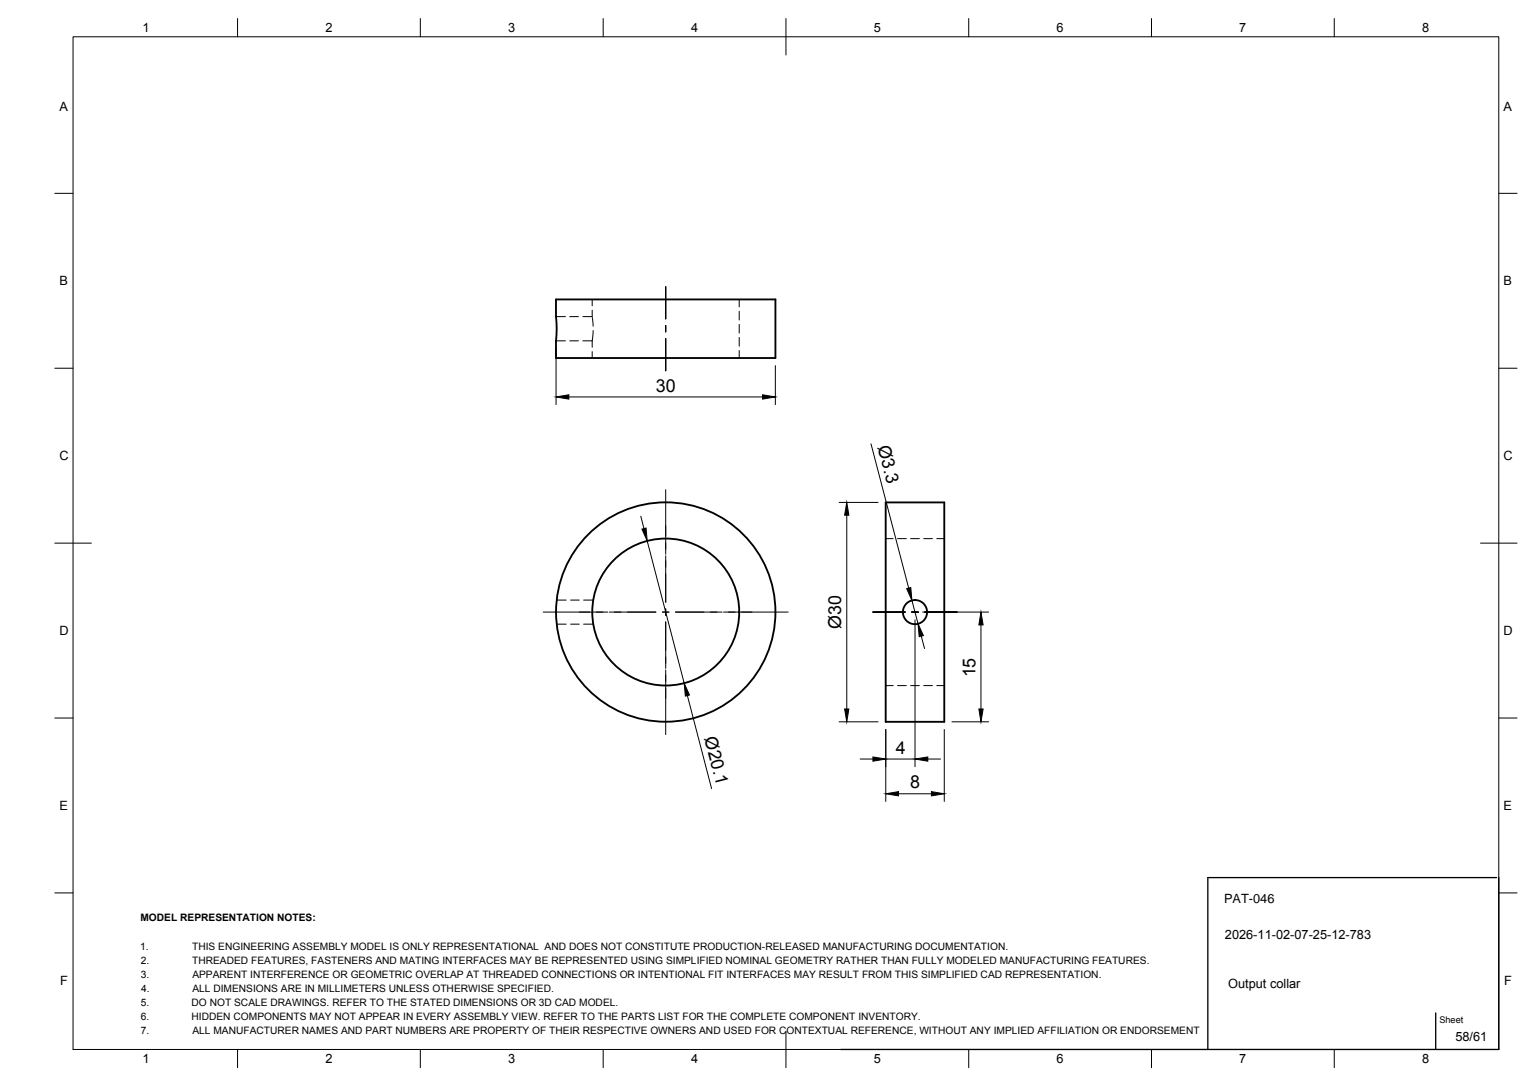
ISO-10303-21;
HEADER;
/* Generated by software containing ST-Developer
 * from STEP Tools, Inc. (www.steptools.com) 
 */

FILE_DESCRIPTION(
/* description */ ('Gear mesh backlash fixture'),
/* implementation_level */ '2;1');

FILE_NAME(
/* name */ 'Output collar.step',
/* time_stamp */ '2026-10-28T03:26:00-07:00',
/* author */ (''),
/* organization */ (''),
/* preprocessor_version */ 'ST-DEVELOPER v20.2',
/* originating_system */ 'Autodesk Translation Framework v15.17.0.0',
/* authorisation */ '');

FILE_SCHEMA (('AUTOMOTIVE_DESIGN { 1 0 10303 214 3 1 1 }'));
ENDSEC;

DATA;
#10=MECHANICAL_DESIGN_GEOMETRIC_PRESENTATION_REPRESENTATION('',(#1075),#57900);
#832=B_SPLINE_CURVE_WITH_KNOTS('',3,(#33907,#33908,#33909,#33910,#33911,
#33912,#33913,#33914,#33915,#33916),.UNSPECIFIED.,.F.,.F.,(4,2,2,2,4),(0.,
0.0622753849594661,0.124550769918932,0.186824589898798,0.249098409878664),
 .UNSPECIFIED.);
#833=B_SPLINE_CURVE_WITH_KNOTS('',3,(#33917,#33918,#33919,#33920,#33921,
#33922,#33923,#33924,#33925,#33926,#33927,#33928,#33929,#33930,#33931,#33932,
#33933,#33934,#33935,#33936,#33937,#33938,#33939,#33940,#33941,#33942),
 .UNSPECIFIED.,.F.,.F.,(4,2,2,2,2,2,2,2,2,2,2,2,4),(0.249098409878664,0.31137222985853,
0.373646049838396,0.435921434797862,0.498196819757329,0.560472204716795,
0.622747589676261,0.685021409656127,0.747295229635993,0.809569049615859,
0.871842869595725,0.934118254555191,0.996393639514657),.UNSPECIFIED.);
#834=B_SPLINE_CURVE_WITH_KNOTS('',3,(#33946,#33947,#33948,#33949,#33950,
#33951,#33952,#33953,#33954,#33955,#33956,#33957,#33958,#33959,#33960,#33961,
#33962,#33963,#33964,#33965,#33966,#33967,#33968,#33969,#33970,#33971),
 .UNSPECIFIED.,.F.,.F.,(4,2,2,2,2,2,2,2,2,2,2,2,4),(0.,0.0622075173149515,
0.124415034629903,0.186622241324509,0.248829448019115,0.311036654713721,
0.373243861408327,0.435451378723279,0.49765889603823,0.559866413353181,
0.622073930668133,0.684281137362739,0.746488344057345),.UNSPECIFIED.);
#835=B_SPLINE_CURVE_WITH_KNOTS('',3,(#33972,#33973,#33974,#33975,#33976,
#33977,#33978,#33979,#33980,#33981),.UNSPECIFIED.,.F.,.F.,(4,2,2,2,4),(0.746488344057345,
0.808695550751951,0.870902757446557,0.933110274761508,0.99531779207646),
 .UNSPECIFIED.);
#960=SHAPE_REPRESENTATION_RELATIONSHIP('SRR','None',#58161,#1010);
#1010=ADVANCED_BREP_SHAPE_REPRESENTATION('',(#1138),#57894);
#1075=STYLED_ITEM('',(#58479),#1138);
#1138=MANIFOLD_SOLID_BREP('Body1',#13637);
#1319=FACE_BOUND('',#3192,.T.);
#1320=FACE_BOUND('',#3194,.T.);
#1321=FACE_BOUND('',#3196,.T.);
#1322=FACE_BOUND('',#3198,.T.);
#1618=PLANE('',#15273);
#1619=PLANE('',#15274);
#2249=FACE_OUTER_BOUND('',#3190,.T.);
#2250=FACE_OUTER_BOUND('',#3191,.T.);
#2251=FACE_OUTER_BOUND('',#3193,.T.);
#2252=FACE_OUTER_BOUND('',#3195,.T.);
#2253=FACE_OUTER_BOUND('',#3197,.T.);
#3190=EDGE_LOOP('',(#11431,#11432,#11433,#11434,#11435,#11436));
#3191=EDGE_LOOP('',(#11437,#11438,#11439,#11440));
#3192=EDGE_LOOP('',(#11441,#11442));
#3193=EDGE_LOOP('',(#11443,#11444,#11445,#11446));
#3194=EDGE_LOOP('',(#11447,#11448));
#3195=EDGE_LOOP('',(#11449));
#3196=EDGE_LOOP('',(#11450));
#3197=EDGE_LOOP('',(#11451));
#3198=EDGE_LOOP('',(#11452));
#4069=LINE('',#33944,#4958);
#4070=LINE('',#33986,#4959);
#4071=LINE('',#33992,#4960);
#4958=VECTOR('',#18380,0.165);
#4959=VECTOR('',#18385,1.005);
#4960=VECTOR('',#18392,1.5);
#5679=CIRCLE('',#15268,1.005);
#5680=CIRCLE('',#15269,1.005);
#5681=CIRCLE('',#15271,1.5);
#5682=CIRCLE('',#15272,1.5);
#6642=VERTEX_POINT('',#33905);
#6643=VERTEX_POINT('',#33906);
#6644=VERTEX_POINT('',#33943);
#6645=VERTEX_POINT('',#33945);
#6646=VERTEX_POINT('',#33983);
#6647=VERTEX_POINT('',#33985);
#6648=VERTEX_POINT('',#33989);
#6649=VERTEX_POINT('',#33991);
#8302=EDGE_CURVE('',#6642,#6643,#832,.T.);
#8303=EDGE_CURVE('',#6643,#6642,#833,.T.);
#8304=EDGE_CURVE('',#6643,#6644,#4069,.T.);
#8305=EDGE_CURVE('',#6645,#6644,#834,.T.);
#8306=EDGE_CURVE('',#6644,#6645,#835,.T.);
#8307=EDGE_CURVE('',#6646,#6646,#5679,.T.);
#8308=EDGE_CURVE('',#6646,#6647,#4070,.T.);
#8309=EDGE_CURVE('',#6647,#6647,#5680,.T.);
#8310=EDGE_CURVE('',#6648,#6648,#5681,.T.);
#8311=EDGE_CURVE('',#6648,#6649,#4071,.T.);
#8312=EDGE_CURVE('',#6649,#6649,#5682,.T.);
#11431=ORIENTED_EDGE('',*,*,#8302,.F.);
#11432=ORIENTED_EDGE('',*,*,#8303,.F.);
#11433=ORIENTED_EDGE('',*,*,#8304,.T.);
#11434=ORIENTED_EDGE('',*,*,#8305,.F.);
#11435=ORIENTED_EDGE('',*,*,#8306,.F.);
#11436=ORIENTED_EDGE('',*,*,#8304,.F.);
#11437=ORIENTED_EDGE('',*,*,#8307,.F.);
#11438=ORIENTED_EDGE('',*,*,#8308,.T.);
#11439=ORIENTED_EDGE('',*,*,#8309,.T.);
#11440=ORIENTED_EDGE('',*,*,#8308,.F.);
#11441=ORIENTED_EDGE('',*,*,#8302,.T.);
#11442=ORIENTED_EDGE('',*,*,#8303,.T.);
#11443=ORIENTED_EDGE('',*,*,#8310,.F.);
#11444=ORIENTED_EDGE('',*,*,#8311,.T.);
#11445=ORIENTED_EDGE('',*,*,#8312,.T.);
#11446=ORIENTED_EDGE('',*,*,#8311,.F.);
#11447=ORIENTED_EDGE('',*,*,#8305,.T.);
#11448=ORIENTED_EDGE('',*,*,#8306,.T.);
#11449=ORIENTED_EDGE('',*,*,#8310,.T.);
#11450=ORIENTED_EDGE('',*,*,#8307,.T.);
#11451=ORIENTED_EDGE('',*,*,#8312,.F.);
#11452=ORIENTED_EDGE('',*,*,#8309,.F.);
#12761=CYLINDRICAL_SURFACE('',#15266,0.165);
#12762=CYLINDRICAL_SURFACE('',#15267,1.005);
#12763=CYLINDRICAL_SURFACE('',#15270,1.5);
#13366=ADVANCED_FACE('',(#2249),#12761,.F.);
#13367=ADVANCED_FACE('',(#2250,#1319),#12762,.F.);
#13368=ADVANCED_FACE('',(#2251,#1320),#12763,.T.);
#13369=ADVANCED_FACE('',(#2252,#1321),#1618,.T.);
#13370=ADVANCED_FACE('',(#2253,#1322),#1619,.F.);
#13637=CLOSED_SHELL('',(#13366,#13367,#13368,#13369,#13370));
#15265=AXIS2_PLACEMENT_3D('',#33903,#18376,#18377);
#15266=AXIS2_PLACEMENT_3D('',#33904,#18378,#18379);
#15267=AXIS2_PLACEMENT_3D('',#33982,#18381,#18382);
#15268=AXIS2_PLACEMENT_3D('',#33984,#18383,#18384);
#15269=AXIS2_PLACEMENT_3D('',#33987,#18386,#18387);
#15270=AXIS2_PLACEMENT_3D('',#33988,#18388,#18389);
#15271=AXIS2_PLACEMENT_3D('',#33990,#18390,#18391);
#15272=AXIS2_PLACEMENT_3D('',#33993,#18393,#18394);
#15273=AXIS2_PLACEMENT_3D('',#33994,#18395,#18396);
#15274=AXIS2_PLACEMENT_3D('',#33995,#18397,#18398);
#18376=DIRECTION('axis',(0.,0.,1.));
#18377=DIRECTION('refdir',(1.,0.,0.));
#18378=DIRECTION('center_axis',(1.,0.,0.));
#18379=DIRECTION('ref_axis',(0.,0.,-1.));
#18380=DIRECTION('',(1.,0.,0.));
#18381=DIRECTION('center_axis',(0.,0.,1.));
#18382=DIRECTION('ref_axis',(1.,0.,0.));
#18383=DIRECTION('center_axis',(0.,0.,-1.));
#18384=DIRECTION('ref_axis',(1.,0.,0.));
#18385=DIRECTION('',(0.,0.,-1.));
#18386=DIRECTION('center_axis',(0.,0.,-1.));
#18387=DIRECTION('ref_axis',(1.,0.,0.));
#18388=DIRECTION('center_axis',(0.,0.,1.));
#18389=DIRECTION('ref_axis',(1.,0.,0.));
#18390=DIRECTION('center_axis',(0.,0.,1.));
#18391=DIRECTION('ref_axis',(1.,0.,0.));
#18392=DIRECTION('',(0.,0.,-1.));
#18393=DIRECTION('center_axis',(0.,0.,1.));
#18394=DIRECTION('ref_axis',(1.,0.,0.));
#18395=DIRECTION('center_axis',(0.,0.,1.));
#18396=DIRECTION('ref_axis',(1.,0.,0.));
#18397=DIRECTION('center_axis',(0.,0.,1.));
#18398=DIRECTION('ref_axis',(1.,0.,0.));
#33903=CARTESIAN_POINT('',(0.,0.,0.));
#33904=CARTESIAN_POINT('Origin',(6.99,0.,5.4));
#33905=CARTESIAN_POINT('',(6.9913626985115,0.165,5.4));
#33906=CARTESIAN_POINT('',(7.005,-1.18380595689425E-17,5.565));
#33907=CARTESIAN_POINT('Ctrl Pts',(6.9913626985115,0.165,5.4));
#33908=CARTESIAN_POINT('Ctrl Pts',(6.9913626985115,0.165,5.42075846165316));
#33909=CARTESIAN_POINT('Ctrl Pts',(6.99208213234536,0.160843707720237,5.44287436269219));
#33910=CARTESIAN_POINT('Ctrl Pts',(6.99466757507705,0.143993298000807,5.48351551009448));
#33911=CARTESIAN_POINT('Ctrl Pts',(6.9964948147884,0.131301190829395,5.50204404696217));
#33912=CARTESIAN_POINT('Ctrl Pts',(6.99991441892026,0.102044414577984,5.53130082321358));
#33913=CARTESIAN_POINT('Ctrl Pts',(7.00173085232892,0.083515719765581,5.54399321874371));
#33914=CARTESIAN_POINT('Ctrl Pts',(7.00429148829838,0.0428740302308134,
5.56084383788794));
#33915=CARTESIAN_POINT('Ctrl Pts',(7.005,0.0207579399932887,5.565));
#33916=CARTESIAN_POINT('Ctrl Pts',(7.005,2.60208521396521E-17,5.565));
#33917=CARTESIAN_POINT('Ctrl Pts',(7.005,-2.08166817117217E-17,5.565));
#33918=CARTESIAN_POINT('Ctrl Pts',(7.005,-0.0207579399932887,5.565));
#33919=CARTESIAN_POINT('Ctrl Pts',(7.00429148829838,-0.0428740302308134,
5.56084383788794));
#33920=CARTESIAN_POINT('Ctrl Pts',(7.00173085232892,-0.083515719765581,
5.54399321874371));
#33921=CARTESIAN_POINT('Ctrl Pts',(6.99991441892026,-0.102044414577984,
5.53130082321358));
#33922=CARTESIAN_POINT('Ctrl Pts',(6.9964948147884,-0.131301190829395,5.50204404696217));
#33923=CARTESIAN_POINT('Ctrl Pts',(6.99466757507705,-0.143993298000807,
5.48351551009448));
#33924=CARTESIAN_POINT('Ctrl Pts',(6.99208213234536,-0.160843707720237,
5.44287436269219));
#33925=CARTESIAN_POINT('Ctrl Pts',(6.9913626985115,-0.165,5.42075846165316));
#33926=CARTESIAN_POINT('Ctrl Pts',(6.9913626985115,-0.165,5.37924153834684));
#33927=CARTESIAN_POINT('Ctrl Pts',(6.99208213234536,-0.160843707720237,
5.35712563730781));
#33928=CARTESIAN_POINT('Ctrl Pts',(6.99466757507705,-0.143993298000807,
5.31648448990552));
#33929=CARTESIAN_POINT('Ctrl Pts',(6.9964948147884,-0.131301190829395,5.29795595303784));
#33930=CARTESIAN_POINT('Ctrl Pts',(6.99991441892026,-0.102044414577984,
5.26869917678642));
#33931=CARTESIAN_POINT('Ctrl Pts',(7.00173085232892,-0.083515719765581,
5.25600678125629));
#33932=CARTESIAN_POINT('Ctrl Pts',(7.00429148829838,-0.0428740302308134,
5.23915616211206));
#33933=CARTESIAN_POINT('Ctrl Pts',(7.005,-0.0207579399932887,5.235));
#33934=CARTESIAN_POINT('Ctrl Pts',(7.005,0.0207579399932886,5.235));
#33935=CARTESIAN_POINT('Ctrl Pts',(7.00429148829838,0.0428740302308133,
5.23915616211206));
#33936=CARTESIAN_POINT('Ctrl Pts',(7.00173085232892,0.0835157197655809,
5.25600678125629));
#33937=CARTESIAN_POINT('Ctrl Pts',(6.99991441892026,0.102044414577984,5.26869917678642));
#33938=CARTESIAN_POINT('Ctrl Pts',(6.9964948147884,0.131301190829395,5.29795595303784));
#33939=CARTESIAN_POINT('Ctrl Pts',(6.99466757507705,0.143993298000807,5.31648448990552));
#33940=CARTESIAN_POINT('Ctrl Pts',(6.99208213234536,0.160843707720237,5.35712563730781));
#33941=CARTESIAN_POINT('Ctrl Pts',(6.9913626985115,0.165,5.37924153834685));
#33942=CARTESIAN_POINT('Ctrl Pts',(6.9913626985115,0.165,5.4));
#33943=CARTESIAN_POINT('',(7.5,-2.02066721859313E-17,5.565));
#33944=CARTESIAN_POINT('',(6.99,-2.02066721859313E-17,5.565));
#33945=CARTESIAN_POINT('',(7.49089738077441,0.165,5.4));
#33946=CARTESIAN_POINT('Ctrl Pts',(7.49089738077441,0.165,5.4));
#33947=CARTESIAN_POINT('Ctrl Pts',(7.49089738077441,0.165,5.37926416089502));
#33948=CARTESIAN_POINT('Ctrl Pts',(7.49137458218466,0.160852499025072,5.35715772909914));
#33949=CARTESIAN_POINT('Ctrl Pts',(7.49309518705251,0.144008447160945,5.31651015506895));
#33950=CARTESIAN_POINT('Ctrl Pts',(7.49431341615514,0.131312810193433,5.29796757240187));
#33951=CARTESIAN_POINT('Ctrl Pts',(7.49659781052538,0.102032500700889,5.26868726290933));
#33952=CARTESIAN_POINT('Ctrl Pts',(7.49781281581157,0.0834898860986566,
5.25599156878035));
#33953=CARTESIAN_POINT('Ctrl Pts',(7.49952603771524,0.042842204593242,5.2391474746158));
#33954=CARTESIAN_POINT('Ctrl Pts',(7.5,0.0207357355648687,5.235));
#33955=CARTESIAN_POINT('Ctrl Pts',(7.5,-0.0207357355648687,5.235));
#33956=CARTESIAN_POINT('Ctrl Pts',(7.49952603771524,-0.042842204593242,
5.2391474746158));
#33957=CARTESIAN_POINT('Ctrl Pts',(7.49781281581157,-0.0834898860986566,
5.25599156878035));
#33958=CARTESIAN_POINT('Ctrl Pts',(7.49659781052538,-0.102032500700889,
5.26868726290933));
#33959=CARTESIAN_POINT('Ctrl Pts',(7.49431341615514,-0.131312810193433,
5.29796757240187));
#33960=CARTESIAN_POINT('Ctrl Pts',(7.49309518705251,-0.144008447160945,
5.31651015506895));
#33961=CARTESIAN_POINT('Ctrl Pts',(7.49137458218466,-0.160852499025072,
5.35715772909914));
#33962=CARTESIAN_POINT('Ctrl Pts',(7.49089738077441,-0.165,5.37926416089502));
#33963=CARTESIAN_POINT('Ctrl Pts',(7.49089738077441,-0.165,5.42073583910498));
#33964=CARTESIAN_POINT('Ctrl Pts',(7.49137458218466,-0.160852499025072,
5.44284227090086));
#33965=CARTESIAN_POINT('Ctrl Pts',(7.49309518705251,-0.144008447160945,
5.48348984493105));
#33966=CARTESIAN_POINT('Ctrl Pts',(7.49431341615514,-0.131312810193433,
5.50203242759813));
#33967=CARTESIAN_POINT('Ctrl Pts',(7.49659781052538,-0.102032500700889,
5.53131273709067));
#33968=CARTESIAN_POINT('Ctrl Pts',(7.49781281581157,-0.0834898860986566,
5.54400843121965));
#33969=CARTESIAN_POINT('Ctrl Pts',(7.49952603771524,-0.042842204593242,
5.5608525253842));
#33970=CARTESIAN_POINT('Ctrl Pts',(7.5,-0.0207357355648688,5.565));
#33971=CARTESIAN_POINT('Ctrl Pts',(7.5,-8.32667268468867E-17,5.565));
#33972=CARTESIAN_POINT('Ctrl Pts',(7.5,4.85722573273506E-17,5.565));
#33973=CARTESIAN_POINT('Ctrl Pts',(7.5,0.0207357355648687,5.565));
#33974=CARTESIAN_POINT('Ctrl Pts',(7.49952603771524,0.0428422045932419,
5.5608525253842));
#33975=CARTESIAN_POINT('Ctrl Pts',(7.49781281581157,0.0834898860986566,
5.54400843121965));
#33976=CARTESIAN_POINT('Ctrl Pts',(7.49659781052538,0.102032500700889,5.53131273709067));
#33977=CARTESIAN_POINT('Ctrl Pts',(7.49431341615514,0.131312810193433,5.50203242759813));
#33978=CARTESIAN_POINT('Ctrl Pts',(7.49309518705251,0.144008447160945,5.48348984493105));
#33979=CARTESIAN_POINT('Ctrl Pts',(7.49137458218466,0.160852499025072,5.44284227090086));
#33980=CARTESIAN_POINT('Ctrl Pts',(7.49089738077441,0.165,5.42073583910498));
#33981=CARTESIAN_POINT('Ctrl Pts',(7.49089738077441,0.165,5.4));
#33982=CARTESIAN_POINT('Origin',(6.,0.,5.));
#33983=CARTESIAN_POINT('',(4.995,-1.23077003314309E-16,5.8));
#33984=CARTESIAN_POINT('Origin',(6.,0.,5.8));
#33985=CARTESIAN_POINT('',(4.995,-1.23077003314309E-16,5.));
#33986=CARTESIAN_POINT('',(4.995,-1.23077003314309E-16,5.));
#33987=CARTESIAN_POINT('Origin',(6.,0.,5.));
#33988=CARTESIAN_POINT('Origin',(6.,0.,5.));
#33989=CARTESIAN_POINT('',(4.5,-1.83697019872103E-16,5.8));
#33990=CARTESIAN_POINT('Origin',(6.,0.,5.8));
#33991=CARTESIAN_POINT('',(4.5,-1.83697019872103E-16,5.));
#33992=CARTESIAN_POINT('',(4.5,-1.83697019872103E-16,5.));
#33993=CARTESIAN_POINT('Origin',(6.,0.,5.));
#33994=CARTESIAN_POINT('Origin',(6.,0.,5.8));
#33995=CARTESIAN_POINT('Origin',(6.,0.,5.));
#57835=UNCERTAINTY_MEASURE_WITH_UNIT(LENGTH_MEASURE(0.001),#57901,
'DISTANCE_ACCURACY_VALUE',
'Maximum model space distance between geometric entities at asserted c
onnectivities');
#57841=UNCERTAINTY_MEASURE_WITH_UNIT(LENGTH_MEASURE(0.001),#57901,
'DISTANCE_ACCURACY_VALUE',
'Maximum model space distance between geometric entities at asserted c
onnectivities');
#57894=(
GEOMETRIC_REPRESENTATION_CONTEXT(3)
GLOBAL_UNCERTAINTY_ASSIGNED_CONTEXT((#57835))
GLOBAL_UNIT_ASSIGNED_CONTEXT((#57901,#57903,#57904))
REPRESENTATION_CONTEXT('','3D')
);
#57900=(
GEOMETRIC_REPRESENTATION_CONTEXT(3)
GLOBAL_UNCERTAINTY_ASSIGNED_CONTEXT((#57841))
GLOBAL_UNIT_ASSIGNED_CONTEXT((#57901,#57903,#57904))
REPRESENTATION_CONTEXT('','3D')
);
#57901=(
LENGTH_UNIT()
NAMED_UNIT(*)
SI_UNIT(.CENTI.,.METRE.)
);
#57903=(
NAMED_UNIT(*)
PLANE_ANGLE_UNIT()
SI_UNIT($,.RADIAN.)
);
#57904=(
NAMED_UNIT(*)
SI_UNIT($,.STERADIAN.)
SOLID_ANGLE_UNIT()
);
#57957=SHAPE_DEFINITION_REPRESENTATION(#58028,#58161);
#58028=PRODUCT_DEFINITION_SHAPE('',$,#58220);
#58161=SHAPE_REPRESENTATION('',(#15265),#57894);
#58167=PRODUCT_DEFINITION_CONTEXT('part definition',#58343,'design');
#58220=PRODUCT_DEFINITION('Output collar','Output collar',#58278,#58167);
#58278=PRODUCT_DEFINITION_FORMATION('',$,#58397);
#58343=APPLICATION_CONTEXT(
'Core Data for Automotive Mechanical Design Process');
#58344=PRODUCT_CONTEXT('part definition',#58343,'mechanical');
#58397=PRODUCT('Output collar','Output collar','Output collar',(#58344));
#58473=COLOUR_RGB('Off White',0.89,0.88,0.83);
#58474=FILL_AREA_STYLE_COLOUR('',#58473);
#58475=FILL_AREA_STYLE('',(#58474));
#58476=SURFACE_STYLE_FILL_AREA(#58475);
#58477=SURFACE_SIDE_STYLE('',(#58476));
#58478=SURFACE_STYLE_USAGE(.BOTH.,#58477);
#58479=PRESENTATION_STYLE_ASSIGNMENT((#58478));
ENDSEC;
END-ISO-10303-21;
